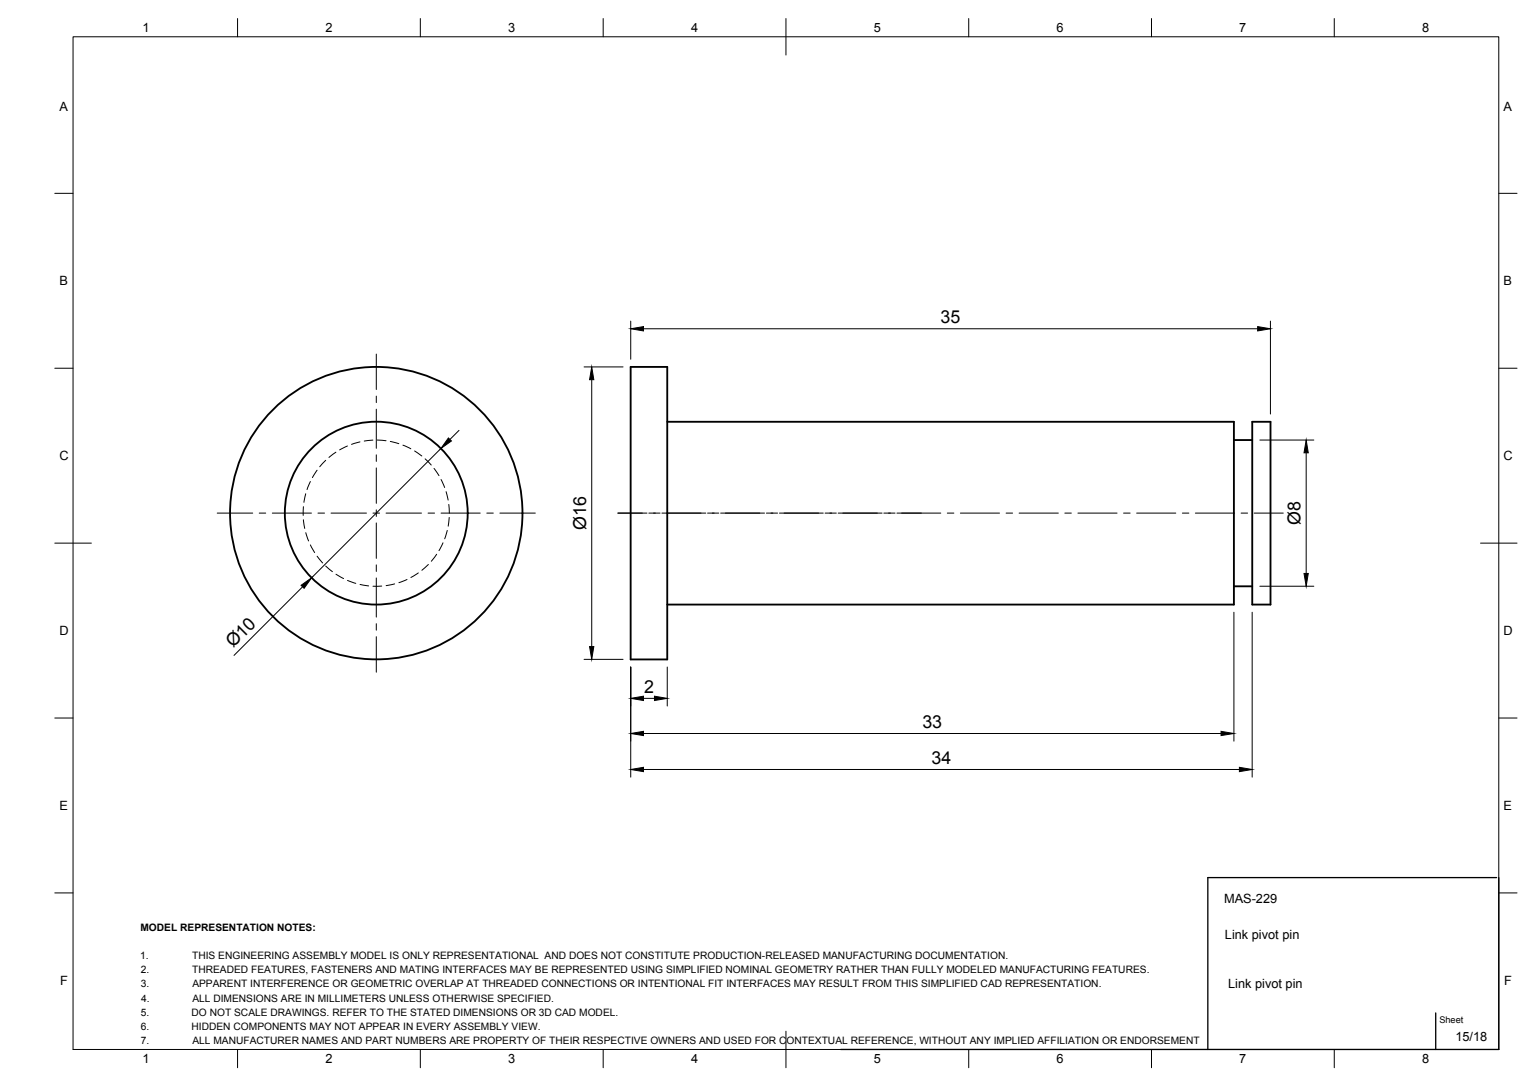
ISO-10303-21;
HEADER;
/* Generated by software containing ST-Developer
 * from STEP Tools, Inc. (www.steptools.com) 
 */

FILE_DESCRIPTION(
/* description */ ('Independently dimensioned six-bar single-leg walking-linkage demonstr
ator. Whole-mm20 crank,60 upper rocker,80/120 ternary coupler,120 lowe
r rocker,140 knee pitch and260 toe reach; ground pivots0/0,60/0,40/60.
 Seven native revolutes close both loops. Four reused native library f
amilies, fully retained shared pins and layered real spacer stacks, bo
nded rubber toe. Benchtop reference mechanism; no complete vehicle, lo
ad, gait stability, adhesive, weld, fit or life rating.'),
/* implementation_level */ '2;1');

FILE_NAME(
/* name */ 'Link pivot pin.step',
/* time_stamp */ '2026-11-09T20:33:14-08:00',
/* author */ (''),
/* organization */ (''),
/* preprocessor_version */ 'ST-DEVELOPER v20.2',
/* originating_system */ 'Autodesk Translation Framework v15.17.0.0',
/* authorisation */ '');

FILE_SCHEMA (('AUTOMOTIVE_DESIGN { 1 0 10303 214 3 1 1 }'));
ENDSEC;

DATA;
#10=MECHANICAL_DESIGN_GEOMETRIC_PRESENTATION_REPRESENTATION('',(#270),#4048);
#234=SHAPE_REPRESENTATION_RELATIONSHIP('SRR','None',#4158,#252);
#252=ADVANCED_BREP_SHAPE_REPRESENTATION('',(#288),#4045);
#270=STYLED_ITEM('',(#4251),#288);
#288=MANIFOLD_SOLID_BREP('Body1',#2159);
#341=FACE_BOUND('',#702,.T.);
#342=FACE_BOUND('',#704,.T.);
#343=FACE_BOUND('',#707,.T.);
#406=PLANE('',#2588);
#407=PLANE('',#2590);
#408=PLANE('',#2594);
#409=PLANE('',#2599);
#410=PLANE('',#2601);
#524=FACE_OUTER_BOUND('',#700,.T.);
#525=FACE_OUTER_BOUND('',#701,.T.);
#526=FACE_OUTER_BOUND('',#703,.T.);
#527=FACE_OUTER_BOUND('',#705,.T.);
#528=FACE_OUTER_BOUND('',#706,.T.);
#529=FACE_OUTER_BOUND('',#708,.T.);
#530=FACE_OUTER_BOUND('',#709,.T.);
#531=FACE_OUTER_BOUND('',#710,.T.);
#532=FACE_OUTER_BOUND('',#711,.T.);
#700=EDGE_LOOP('',(#1915,#1916,#1917,#1918));
#701=EDGE_LOOP('',(#1919));
#702=EDGE_LOOP('',(#1920));
#703=EDGE_LOOP('',(#1921));
#704=EDGE_LOOP('',(#1922));
#705=EDGE_LOOP('',(#1923,#1924,#1925,#1926));
#706=EDGE_LOOP('',(#1927));
#707=EDGE_LOOP('',(#1928));
#708=EDGE_LOOP('',(#1929,#1930,#1931,#1932));
#709=EDGE_LOOP('',(#1933));
#710=EDGE_LOOP('',(#1934,#1935,#1936,#1937));
#711=EDGE_LOOP('',(#1938));
#841=LINE('',#3903,#966);
#842=LINE('',#3914,#967);
#843=LINE('',#3922,#968);
#844=LINE('',#3926,#969);
#966=VECTOR('',#3240,4.);
#967=VECTOR('',#3255,5.);
#968=VECTOR('',#3264,8.);
#969=VECTOR('',#3271,5.);
#1072=CIRCLE('',#2586,4.);
#1073=CIRCLE('',#2587,4.);
#1074=CIRCLE('',#2589,5.);
#1075=CIRCLE('',#2591,5.);
#1076=CIRCLE('',#2593,5.);
#1077=CIRCLE('',#2595,8.);
#1078=CIRCLE('',#2596,5.);
#1079=CIRCLE('',#2598,8.);
#1230=VERTEX_POINT('',#3900);
#1231=VERTEX_POINT('',#3902);
#1232=VERTEX_POINT('',#3906);
#1233=VERTEX_POINT('',#3909);
#1234=VERTEX_POINT('',#3912);
#1235=VERTEX_POINT('',#3916);
#1236=VERTEX_POINT('',#3918);
#1237=VERTEX_POINT('',#3921);
#1461=EDGE_CURVE('',#1230,#1230,#1072,.T.);
#1462=EDGE_CURVE('',#1230,#1231,#841,.T.);
#1463=EDGE_CURVE('',#1231,#1231,#1073,.T.);
#1464=EDGE_CURVE('',#1232,#1232,#1074,.T.);
#1465=EDGE_CURVE('',#1233,#1233,#1075,.T.);
#1466=EDGE_CURVE('',#1234,#1234,#1076,.T.);
#1467=EDGE_CURVE('',#1234,#1233,#842,.T.);
#1468=EDGE_CURVE('',#1235,#1235,#1077,.T.);
#1469=EDGE_CURVE('',#1236,#1236,#1078,.T.);
#1470=EDGE_CURVE('',#1235,#1237,#843,.T.);
#1471=EDGE_CURVE('',#1237,#1237,#1079,.T.);
#1472=EDGE_CURVE('',#1232,#1236,#844,.T.);
#1915=ORIENTED_EDGE('',*,*,#1461,.T.);
#1916=ORIENTED_EDGE('',*,*,#1462,.T.);
#1917=ORIENTED_EDGE('',*,*,#1463,.F.);
#1918=ORIENTED_EDGE('',*,*,#1462,.F.);
#1919=ORIENTED_EDGE('',*,*,#1464,.F.);
#1920=ORIENTED_EDGE('',*,*,#1461,.F.);
#1921=ORIENTED_EDGE('',*,*,#1465,.F.);
#1922=ORIENTED_EDGE('',*,*,#1463,.T.);
#1923=ORIENTED_EDGE('',*,*,#1466,.F.);
#1924=ORIENTED_EDGE('',*,*,#1467,.T.);
#1925=ORIENTED_EDGE('',*,*,#1465,.T.);
#1926=ORIENTED_EDGE('',*,*,#1467,.F.);
#1927=ORIENTED_EDGE('',*,*,#1468,.T.);
#1928=ORIENTED_EDGE('',*,*,#1469,.F.);
#1929=ORIENTED_EDGE('',*,*,#1468,.F.);
#1930=ORIENTED_EDGE('',*,*,#1470,.T.);
#1931=ORIENTED_EDGE('',*,*,#1471,.T.);
#1932=ORIENTED_EDGE('',*,*,#1470,.F.);
#1933=ORIENTED_EDGE('',*,*,#1471,.F.);
#1934=ORIENTED_EDGE('',*,*,#1464,.T.);
#1935=ORIENTED_EDGE('',*,*,#1472,.T.);
#1936=ORIENTED_EDGE('',*,*,#1469,.T.);
#1937=ORIENTED_EDGE('',*,*,#1472,.F.);
#1938=ORIENTED_EDGE('',*,*,#1466,.T.);
#2010=CYLINDRICAL_SURFACE('',#2585,4.);
#2011=CYLINDRICAL_SURFACE('',#2592,5.);
#2012=CYLINDRICAL_SURFACE('',#2597,8.);
#2013=CYLINDRICAL_SURFACE('',#2600,5.);
#2127=ADVANCED_FACE('',(#524),#2010,.T.);
#2128=ADVANCED_FACE('',(#525,#341),#406,.F.);
#2129=ADVANCED_FACE('',(#526,#342),#407,.F.);
#2130=ADVANCED_FACE('',(#527),#2011,.T.);
#2131=ADVANCED_FACE('',(#528,#343),#408,.T.);
#2132=ADVANCED_FACE('',(#529),#2012,.T.);
#2133=ADVANCED_FACE('',(#530),#409,.F.);
#2134=ADVANCED_FACE('',(#531),#2013,.T.);
#2135=ADVANCED_FACE('',(#532),#410,.T.);
#2159=CLOSED_SHELL('',(#2127,#2128,#2129,#2130,#2131,#2132,#2133,#2134,
#2135));
#2584=AXIS2_PLACEMENT_3D('',#3898,#3234,#3235);
#2585=AXIS2_PLACEMENT_3D('',#3899,#3236,#3237);
#2586=AXIS2_PLACEMENT_3D('',#3901,#3238,#3239);
#2587=AXIS2_PLACEMENT_3D('',#3904,#3241,#3242);
#2588=AXIS2_PLACEMENT_3D('',#3905,#3243,#3244);
#2589=AXIS2_PLACEMENT_3D('',#3907,#3245,#3246);
#2590=AXIS2_PLACEMENT_3D('',#3908,#3247,#3248);
#2591=AXIS2_PLACEMENT_3D('',#3910,#3249,#3250);
#2592=AXIS2_PLACEMENT_3D('',#3911,#3251,#3252);
#2593=AXIS2_PLACEMENT_3D('',#3913,#3253,#3254);
#2594=AXIS2_PLACEMENT_3D('',#3915,#3256,#3257);
#2595=AXIS2_PLACEMENT_3D('',#3917,#3258,#3259);
#2596=AXIS2_PLACEMENT_3D('',#3919,#3260,#3261);
#2597=AXIS2_PLACEMENT_3D('',#3920,#3262,#3263);
#2598=AXIS2_PLACEMENT_3D('',#3923,#3265,#3266);
#2599=AXIS2_PLACEMENT_3D('',#3924,#3267,#3268);
#2600=AXIS2_PLACEMENT_3D('',#3925,#3269,#3270);
#2601=AXIS2_PLACEMENT_3D('',#3927,#3272,#3273);
#3234=DIRECTION('axis',(0.,0.,1.));
#3235=DIRECTION('refdir',(1.,0.,0.));
#3236=DIRECTION('center_axis',(0.,0.,1.));
#3237=DIRECTION('ref_axis',(1.,0.,0.));
#3238=DIRECTION('center_axis',(0.,0.,1.));
#3239=DIRECTION('ref_axis',(1.,0.,0.));
#3240=DIRECTION('',(0.,0.,1.));
#3241=DIRECTION('center_axis',(0.,0.,1.));
#3242=DIRECTION('ref_axis',(1.,0.,0.));
#3243=DIRECTION('center_axis',(0.,0.,-1.));
#3244=DIRECTION('ref_axis',(-1.,0.,0.));
#3245=DIRECTION('center_axis',(0.,0.,-1.));
#3246=DIRECTION('ref_axis',(1.,0.,0.));
#3247=DIRECTION('center_axis',(0.,0.,1.));
#3248=DIRECTION('ref_axis',(1.,0.,0.));
#3249=DIRECTION('center_axis',(0.,0.,1.));
#3250=DIRECTION('ref_axis',(1.,0.,0.));
#3251=DIRECTION('center_axis',(0.,0.,1.));
#3252=DIRECTION('ref_axis',(1.,0.,0.));
#3253=DIRECTION('center_axis',(0.,0.,1.));
#3254=DIRECTION('ref_axis',(1.,0.,0.));
#3255=DIRECTION('',(0.,0.,-1.));
#3256=DIRECTION('center_axis',(0.,0.,1.));
#3257=DIRECTION('ref_axis',(1.,0.,0.));
#3258=DIRECTION('center_axis',(0.,0.,1.));
#3259=DIRECTION('ref_axis',(1.,0.,0.));
#3260=DIRECTION('center_axis',(0.,0.,1.));
#3261=DIRECTION('ref_axis',(1.,0.,0.));
#3262=DIRECTION('center_axis',(0.,0.,1.));
#3263=DIRECTION('ref_axis',(1.,0.,0.));
#3264=DIRECTION('',(0.,0.,-1.));
#3265=DIRECTION('center_axis',(0.,0.,1.));
#3266=DIRECTION('ref_axis',(1.,0.,0.));
#3267=DIRECTION('center_axis',(0.,0.,1.));
#3268=DIRECTION('ref_axis',(1.,0.,0.));
#3269=DIRECTION('center_axis',(0.,0.,1.));
#3270=DIRECTION('ref_axis',(1.,0.,0.));
#3271=DIRECTION('',(0.,0.,-1.));
#3272=DIRECTION('center_axis',(0.,0.,1.));
#3273=DIRECTION('ref_axis',(1.,0.,0.));
#3898=CARTESIAN_POINT('',(0.,0.,0.));
#3899=CARTESIAN_POINT('Origin',(0.,0.,31.5));
#3900=CARTESIAN_POINT('',(-4.,-4.89858719658941E-16,31.));
#3901=CARTESIAN_POINT('Origin',(0.,0.,31.));
#3902=CARTESIAN_POINT('',(-4.,-4.89858719658941E-16,32.));
#3903=CARTESIAN_POINT('',(-4.,-4.89858719658941E-16,31.5));
#3904=CARTESIAN_POINT('Origin',(0.,0.,32.));
#3905=CARTESIAN_POINT('Origin',(8.,0.,31.));
#3906=CARTESIAN_POINT('',(-5.,6.12323399573677E-16,31.));
#3907=CARTESIAN_POINT('Origin',(0.,0.,31.));
#3908=CARTESIAN_POINT('Origin',(4.,0.,32.));
#3909=CARTESIAN_POINT('',(-5.,-6.12323399573677E-16,32.));
#3910=CARTESIAN_POINT('Origin',(0.,0.,32.));
#3911=CARTESIAN_POINT('Origin',(0.,0.,0.));
#3912=CARTESIAN_POINT('',(-5.,-6.12323399573677E-16,33.));
#3913=CARTESIAN_POINT('Origin',(0.,0.,33.));
#3914=CARTESIAN_POINT('',(-5.,-6.12323399573677E-16,0.));
#3915=CARTESIAN_POINT('Origin',(0.,0.,0.));
#3916=CARTESIAN_POINT('',(-8.,-9.79717439317883E-16,0.));
#3917=CARTESIAN_POINT('Origin',(0.,0.,0.));
#3918=CARTESIAN_POINT('',(-5.,-6.12323399573677E-16,0.));
#3919=CARTESIAN_POINT('Origin',(0.,0.,0.));
#3920=CARTESIAN_POINT('Origin',(0.,0.,-2.));
#3921=CARTESIAN_POINT('',(-8.,-9.79717439317883E-16,-2.));
#3922=CARTESIAN_POINT('',(-8.,-9.79717439317883E-16,-2.));
#3923=CARTESIAN_POINT('Origin',(0.,0.,-2.));
#3924=CARTESIAN_POINT('Origin',(0.,0.,-2.));
#3925=CARTESIAN_POINT('Origin',(0.,0.,0.));
#3926=CARTESIAN_POINT('',(-5.,-6.12323399573677E-16,0.));
#3927=CARTESIAN_POINT('Origin',(0.,0.,33.));
#4025=UNCERTAINTY_MEASURE_WITH_UNIT(LENGTH_MEASURE(0.01),#4049,
'DISTANCE_ACCURACY_VALUE',
'Maximum model space distance between geometric entities at asserted c
onnectivities');
#4028=UNCERTAINTY_MEASURE_WITH_UNIT(LENGTH_MEASURE(0.01),#4049,
'DISTANCE_ACCURACY_VALUE',
'Maximum model space distance between geometric entities at asserted c
onnectivities');
#4045=(
GEOMETRIC_REPRESENTATION_CONTEXT(3)
GLOBAL_UNCERTAINTY_ASSIGNED_CONTEXT((#4025))
GLOBAL_UNIT_ASSIGNED_CONTEXT((#4049,#4051,#4052))
REPRESENTATION_CONTEXT('','3D')
);
#4048=(
GEOMETRIC_REPRESENTATION_CONTEXT(3)
GLOBAL_UNCERTAINTY_ASSIGNED_CONTEXT((#4028))
GLOBAL_UNIT_ASSIGNED_CONTEXT((#4049,#4051,#4052))
REPRESENTATION_CONTEXT('','3D')
);
#4049=(
LENGTH_UNIT()
NAMED_UNIT(*)
SI_UNIT(.MILLI.,.METRE.)
);
#4051=(
NAMED_UNIT(*)
PLANE_ANGLE_UNIT()
SI_UNIT($,.RADIAN.)
);
#4052=(
NAMED_UNIT(*)
SI_UNIT($,.STERADIAN.)
SOLID_ANGLE_UNIT()
);
#4069=SHAPE_DEFINITION_REPRESENTATION(#4088,#4158);
#4088=PRODUCT_DEFINITION_SHAPE('',$,#4178);
#4158=SHAPE_REPRESENTATION('',(#2584),#4045);
#4161=PRODUCT_DEFINITION_CONTEXT('part definition',#4220,'design');
#4178=PRODUCT_DEFINITION('Link pivot pin','Link pivot pin',#4197,#4161);
#4197=PRODUCT_DEFINITION_FORMATION('',$,#4238);
#4220=APPLICATION_CONTEXT(
'Core Data for Automotive Mechanical Design Process');
#4221=PRODUCT_CONTEXT('part definition',#4220,'mechanical');
#4238=PRODUCT('Link pivot pin','Link pivot pin',$,(#4221));
#4251=PRESENTATION_STYLE_ASSIGNMENT((#4265));
#4265=SURFACE_STYLE_USAGE(.BOTH.,#4279);
#4279=SURFACE_SIDE_STYLE('',(#4293));
#4293=SURFACE_STYLE_FILL_AREA(#4307);
#4307=FILL_AREA_STYLE('Pin gray',(#4321));
#4321=FILL_AREA_STYLE_COLOUR('Pin gray',#4335);
#4335=COLOUR_RGB('Pin gray',0.576470588235294,0.615686274509804,0.666666666666667);
ENDSEC;
END-ISO-10303-21;
